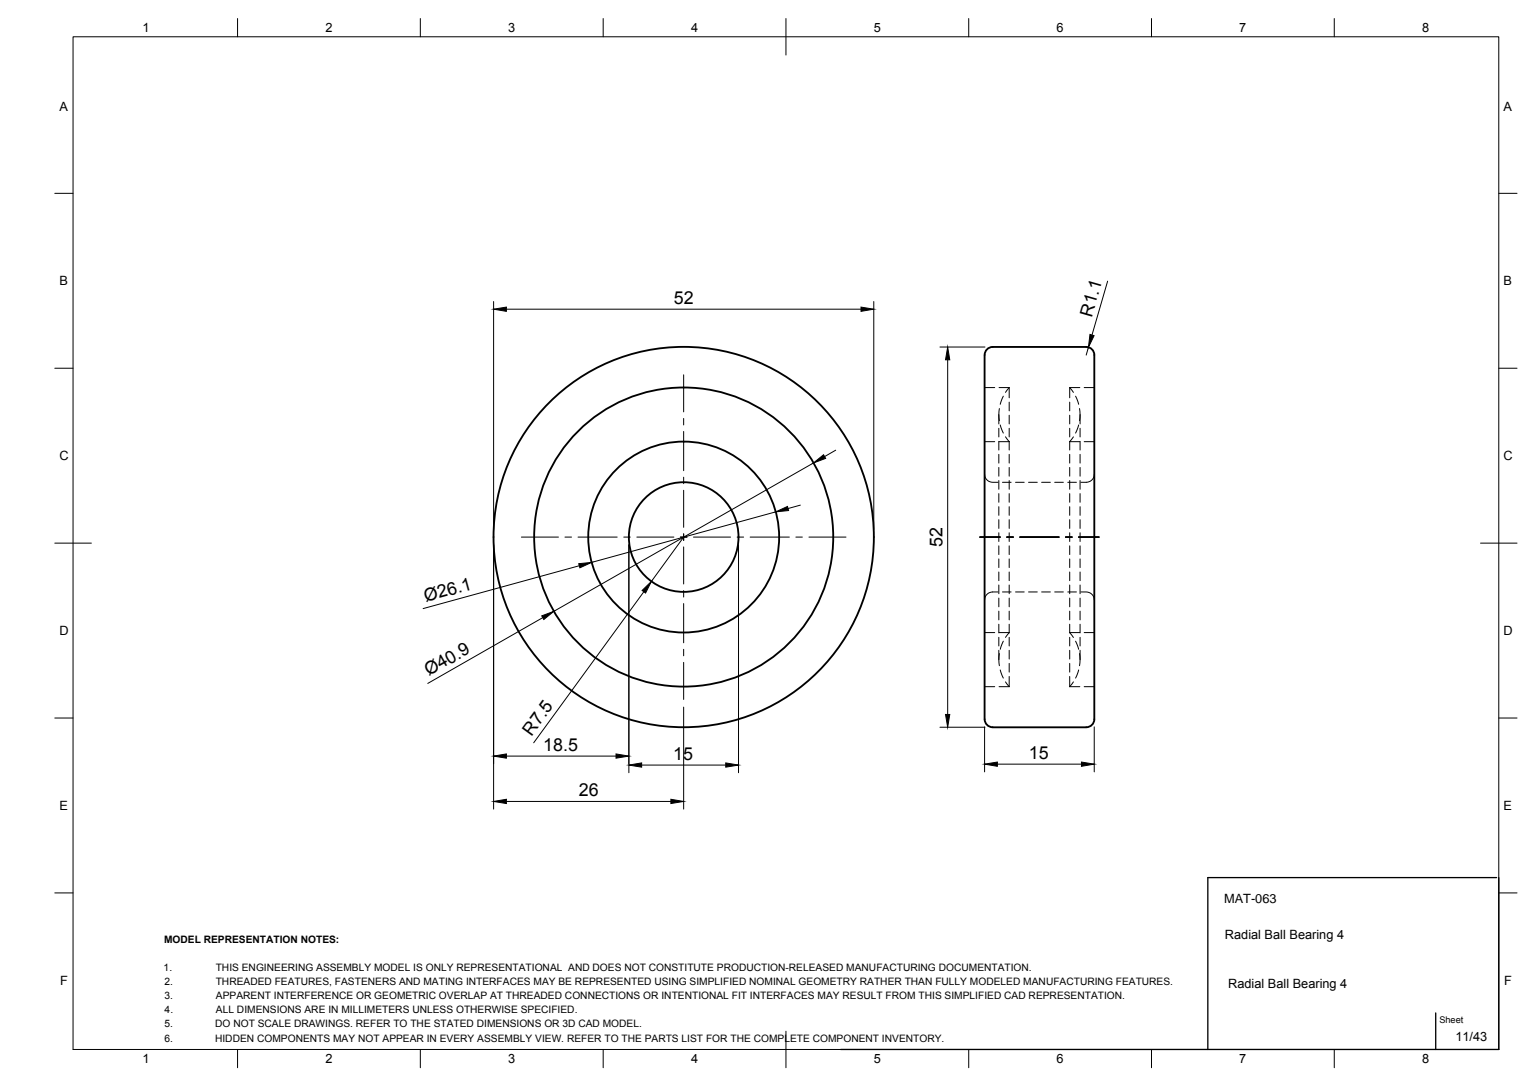
ISO-10303-21;
HEADER;
/* Generated by software containing ST-Developer
 * from STEP Tools, Inc. (www.steptools.com) 
 */

FILE_DESCRIPTION(
/* description */ (''),
/* implementation_level */ '2;1');

FILE_NAME(
/* name */ 'Radial Ball Bearing 4.step',
/* time_stamp */ '2026-10-24T09:43:01-07:00',
/* author */ (''),
/* organization */ (''),
/* preprocessor_version */ 'ST-DEVELOPER v20.2',
/* originating_system */ 'Autodesk Translation Framework v15.15.0.0',
/* authorisation */ '');

FILE_SCHEMA (('AUTOMOTIVE_DESIGN { 1 0 10303 214 3 1 1 }'));
ENDSEC;

DATA;
#10=MECHANICAL_DESIGN_GEOMETRIC_PRESENTATION_REPRESENTATION('',(#281),#11112);
#197=TOROIDAL_SURFACE('',#6769,0.0248999989285722,0.00110000131901909);
#198=TOROIDAL_SURFACE('',#6774,0.0248999989285722,0.00110000131901909);
#199=TOROIDAL_SURFACE('',#6782,0.0248999989285722,0.00110000131901911);
#200=TOROIDAL_SURFACE('',#6789,0.0248999989285722,0.00110000131901911);
#201=TOROIDAL_SURFACE('',#6793,0.01675,0.00555000054498457);
#202=TOROIDAL_SURFACE('',#6802,0.01675,0.00555000054498457);
#203=TOROIDAL_SURFACE('',#6811,0.00860000107142784,0.00110000131901912);
#204=TOROIDAL_SURFACE('',#6815,0.00860000107142784,0.00110000131901912);
#205=TOROIDAL_SURFACE('',#6823,0.00860000107142785,0.00110000131901912);
#206=TOROIDAL_SURFACE('',#6826,0.00860000107142785,0.00110000131901912);
#215=SHAPE_REPRESENTATION_RELATIONSHIP('SRR','None',#11238,#248);
#248=ADVANCED_BREP_SHAPE_REPRESENTATION('',(#314),#11083);
#281=STYLED_ITEM('',(#11425),#314);
#314=MANIFOLD_SOLID_BREP('Radial Ball Bearing 4',#6018);
#408=FACE_BOUND('',#1254,.T.);
#409=FACE_BOUND('',#1259,.T.);
#410=FACE_BOUND('',#1265,.T.);
#411=FACE_BOUND('',#1270,.T.);
#539=PLANE('',#6780);
#540=PLANE('',#6791);
#541=PLANE('',#6806);
#542=PLANE('',#6817);
#817=FACE_OUTER_BOUND('',#1250,.T.);
#818=FACE_OUTER_BOUND('',#1251,.T.);
#819=FACE_OUTER_BOUND('',#1252,.T.);
#820=FACE_OUTER_BOUND('',#1253,.T.);
#821=FACE_OUTER_BOUND('',#1255,.T.);
#822=FACE_OUTER_BOUND('',#1256,.T.);
#823=FACE_OUTER_BOUND('',#1257,.T.);
#824=FACE_OUTER_BOUND('',#1258,.T.);
#825=FACE_OUTER_BOUND('',#1260,.T.);
#826=FACE_OUTER_BOUND('',#1261,.T.);
#827=FACE_OUTER_BOUND('',#1262,.T.);
#828=FACE_OUTER_BOUND('',#1263,.T.);
#829=FACE_OUTER_BOUND('',#1264,.T.);
#830=FACE_OUTER_BOUND('',#1266,.T.);
#831=FACE_OUTER_BOUND('',#1267,.T.);
#832=FACE_OUTER_BOUND('',#1268,.T.);
#833=FACE_OUTER_BOUND('',#1269,.T.);
#834=FACE_OUTER_BOUND('',#1271,.T.);
#835=FACE_OUTER_BOUND('',#1272,.T.);
#836=FACE_OUTER_BOUND('',#1273,.T.);
#1250=EDGE_LOOP('',(#4579,#4580,#4581,#4582));
#1251=EDGE_LOOP('',(#4583,#4584,#4585,#4586));
#1252=EDGE_LOOP('',(#4587,#4588,#4589,#4590,#4591,#4592));
#1253=EDGE_LOOP('',(#4593,#4594));
#1254=EDGE_LOOP('',(#4595));
#1255=EDGE_LOOP('',(#4596,#4597,#4598,#4599));
#1256=EDGE_LOOP('',(#4600,#4601,#4602,#4603,#4604));
#1257=EDGE_LOOP('',(#4605,#4606,#4607,#4608));
#1258=EDGE_LOOP('',(#4609,#4610));
#1259=EDGE_LOOP('',(#4611));
#1260=EDGE_LOOP('',(#4612,#4613,#4614,#4615,#4616,#4617));
#1261=EDGE_LOOP('',(#4618,#4619,#4620,#4621,#4622));
#1262=EDGE_LOOP('',(#4623,#4624,#4625,#4626,#4627));
#1263=EDGE_LOOP('',(#4628,#4629,#4630,#4631,#4632,#4633));
#1264=EDGE_LOOP('',(#4634));
#1265=EDGE_LOOP('',(#4635,#4636));
#1266=EDGE_LOOP('',(#4637,#4638,#4639,#4640,#4641));
#1267=EDGE_LOOP('',(#4642,#4643,#4644,#4645));
#1268=EDGE_LOOP('',(#4646,#4647,#4648,#4649));
#1269=EDGE_LOOP('',(#4650));
#1270=EDGE_LOOP('',(#4651,#4652));
#1271=EDGE_LOOP('',(#4653,#4654,#4655,#4656,#4657,#4658));
#1272=EDGE_LOOP('',(#4659,#4660,#4661,#4662));
#1273=EDGE_LOOP('',(#4663,#4664,#4665,#4666));
#1663=LINE('',#10007,#2022);
#1664=LINE('',#10019,#2023);
#1665=LINE('',#10039,#2024);
#1666=LINE('',#10042,#2025);
#1667=LINE('',#10058,#2026);
#1668=LINE('',#10074,#2027);
#2022=VECTOR('',#8111,0.026);
#2023=VECTOR('',#8126,0.02045);
#2024=VECTOR('',#8153,0.02045);
#2025=VECTOR('',#8156,0.01305);
#2026=VECTOR('',#8177,0.01305);
#2027=VECTOR('',#8198,0.0075);
#2484=CIRCLE('',#6770,0.0248999997701383);
#2485=CIRCLE('',#6771,0.00110000131901909);
#2486=CIRCLE('',#6772,0.0260000002475909);
#2487=CIRCLE('',#6773,0.00110000131901909);
#2488=CIRCLE('',#6775,0.0248999997701383);
#2489=CIRCLE('',#6776,0.0260000002475909);
#2490=CIRCLE('',#6778,0.026);
#2491=CIRCLE('',#6779,0.026);
#2492=CIRCLE('',#6781,0.02045);
#2493=CIRCLE('',#6783,0.00110000131901911);
#2494=CIRCLE('',#6784,0.0248999997701383);
#2495=CIRCLE('',#6785,0.0011000013190191);
#2496=CIRCLE('',#6787,0.02045);
#2497=CIRCLE('',#6788,0.02045);
#2498=CIRCLE('',#6790,0.0248999997701383);
#2499=CIRCLE('',#6792,0.02045);
#2500=CIRCLE('',#6794,0.00555000054498457);
#2501=CIRCLE('',#6795,0.0130499999271107);
#2502=CIRCLE('',#6796,0.0130499999271107);
#2503=CIRCLE('',#6798,0.02045);
#2504=CIRCLE('',#6799,0.02045);
#2505=CIRCLE('',#6801,0.01305);
#2506=CIRCLE('',#6803,0.01305);
#2507=CIRCLE('',#6804,0.00555000054498457);
#2508=CIRCLE('',#6805,0.01305);
#2509=CIRCLE('',#6807,0.00860000022986177);
#2510=CIRCLE('',#6808,0.00860000022986177);
#2511=CIRCLE('',#6810,0.01305);
#2512=CIRCLE('',#6812,0.00110000131901912);
#2513=CIRCLE('',#6813,0.00749999975240907);
#2514=CIRCLE('',#6814,0.00110000131901912);
#2515=CIRCLE('',#6816,0.00749999975240873);
#2516=CIRCLE('',#6818,0.00860000022986177);
#2517=CIRCLE('',#6819,0.00860000022986177);
#2518=CIRCLE('',#6821,0.0075);
#2519=CIRCLE('',#6822,0.00749999975240873);
#2520=CIRCLE('',#6824,0.00110000131901912);
#2521=CIRCLE('',#6825,0.00110000131901912);
#2880=VERTEX_POINT('',#9991);
#2881=VERTEX_POINT('',#9992);
#2882=VERTEX_POINT('',#9994);
#2883=VERTEX_POINT('',#9996);
#2884=VERTEX_POINT('',#10003);
#2885=VERTEX_POINT('',#10004);
#2886=VERTEX_POINT('',#10009);
#2887=VERTEX_POINT('',#10012);
#2888=VERTEX_POINT('',#10014);
#2889=VERTEX_POINT('',#10018);
#2890=VERTEX_POINT('',#10020);
#2891=VERTEX_POINT('',#10026);
#2892=VERTEX_POINT('',#10029);
#2893=VERTEX_POINT('',#10031);
#2894=VERTEX_POINT('',#10035);
#2895=VERTEX_POINT('',#10036);
#2896=VERTEX_POINT('',#10041);
#2897=VERTEX_POINT('',#10045);
#2898=VERTEX_POINT('',#10046);
#2899=VERTEX_POINT('',#10051);
#2900=VERTEX_POINT('',#10052);
#2901=VERTEX_POINT('',#10056);
#2902=VERTEX_POINT('',#10060);
#2903=VERTEX_POINT('',#10062);
#2904=VERTEX_POINT('',#10068);
#2905=VERTEX_POINT('',#10069);
#2906=VERTEX_POINT('',#10073);
#2907=VERTEX_POINT('',#10075);
#3493=EDGE_CURVE('',#2880,#2881,#2484,.T.);
#3494=EDGE_CURVE('',#2881,#2882,#2485,.T.);
#3495=EDGE_CURVE('',#2882,#2883,#2486,.F.);
#3496=EDGE_CURVE('',#2883,#2880,#2487,.T.);
#3497=EDGE_CURVE('',#2881,#2880,#2488,.T.);
#3498=EDGE_CURVE('',#2883,#2882,#2489,.T.);
#3499=EDGE_CURVE('',#2884,#2885,#2490,.F.);
#3500=EDGE_CURVE('',#2885,#2884,#2491,.F.);
#3501=EDGE_CURVE('',#2884,#2882,#1663,.T.);
#3502=EDGE_CURVE('',#2886,#2886,#2492,.T.);
#3503=EDGE_CURVE('',#2884,#2887,#2493,.T.);
#3504=EDGE_CURVE('',#2887,#2888,#2494,.F.);
#3505=EDGE_CURVE('',#2888,#2885,#2495,.T.);
#3506=EDGE_CURVE('',#2886,#2889,#1664,.T.);
#3507=EDGE_CURVE('',#2890,#2889,#2496,.F.);
#3508=EDGE_CURVE('',#2889,#2890,#2497,.F.);
#3509=EDGE_CURVE('',#2888,#2887,#2498,.F.);
#3510=EDGE_CURVE('',#2891,#2891,#2499,.F.);
#3511=EDGE_CURVE('',#2890,#2892,#2500,.T.);
#3512=EDGE_CURVE('',#2892,#2893,#2501,.T.);
#3513=EDGE_CURVE('',#2893,#2892,#2502,.T.);
#3514=EDGE_CURVE('',#2894,#2895,#2503,.F.);
#3515=EDGE_CURVE('',#2895,#2894,#2504,.F.);
#3516=EDGE_CURVE('',#2895,#2891,#1665,.T.);
#3517=EDGE_CURVE('',#2893,#2896,#1666,.T.);
#3518=EDGE_CURVE('',#2896,#2896,#2505,.T.);
#3519=EDGE_CURVE('',#2897,#2898,#2506,.T.);
#3520=EDGE_CURVE('',#2898,#2894,#2507,.T.);
#3521=EDGE_CURVE('',#2898,#2897,#2508,.T.);
#3522=EDGE_CURVE('',#2899,#2900,#2509,.T.);
#3523=EDGE_CURVE('',#2900,#2899,#2510,.T.);
#3524=EDGE_CURVE('',#2901,#2901,#2511,.F.);
#3525=EDGE_CURVE('',#2901,#2897,#1667,.T.);
#3526=EDGE_CURVE('',#2900,#2902,#2512,.T.);
#3527=EDGE_CURVE('',#2902,#2903,#2513,.T.);
#3528=EDGE_CURVE('',#2903,#2899,#2514,.T.);
#3529=EDGE_CURVE('',#2903,#2902,#2515,.T.);
#3530=EDGE_CURVE('',#2904,#2905,#2516,.F.);
#3531=EDGE_CURVE('',#2905,#2904,#2517,.F.);
#3532=EDGE_CURVE('',#2902,#2906,#1668,.T.);
#3533=EDGE_CURVE('',#2907,#2906,#2518,.F.);
#3534=EDGE_CURVE('',#2906,#2907,#2519,.F.);
#3535=EDGE_CURVE('',#2906,#2904,#2520,.T.);
#3536=EDGE_CURVE('',#2905,#2907,#2521,.T.);
#4579=ORIENTED_EDGE('',*,*,#3493,.T.);
#4580=ORIENTED_EDGE('',*,*,#3494,.T.);
#4581=ORIENTED_EDGE('',*,*,#3495,.T.);
#4582=ORIENTED_EDGE('',*,*,#3496,.T.);
#4583=ORIENTED_EDGE('',*,*,#3494,.F.);
#4584=ORIENTED_EDGE('',*,*,#3497,.T.);
#4585=ORIENTED_EDGE('',*,*,#3496,.F.);
#4586=ORIENTED_EDGE('',*,*,#3498,.T.);
#4587=ORIENTED_EDGE('',*,*,#3499,.T.);
#4588=ORIENTED_EDGE('',*,*,#3500,.T.);
#4589=ORIENTED_EDGE('',*,*,#3501,.T.);
#4590=ORIENTED_EDGE('',*,*,#3498,.F.);
#4591=ORIENTED_EDGE('',*,*,#3495,.F.);
#4592=ORIENTED_EDGE('',*,*,#3501,.F.);
#4593=ORIENTED_EDGE('',*,*,#3493,.F.);
#4594=ORIENTED_EDGE('',*,*,#3497,.F.);
#4595=ORIENTED_EDGE('',*,*,#3502,.T.);
#4596=ORIENTED_EDGE('',*,*,#3499,.F.);
#4597=ORIENTED_EDGE('',*,*,#3503,.T.);
#4598=ORIENTED_EDGE('',*,*,#3504,.T.);
#4599=ORIENTED_EDGE('',*,*,#3505,.T.);
#4600=ORIENTED_EDGE('',*,*,#3502,.F.);
#4601=ORIENTED_EDGE('',*,*,#3506,.T.);
#4602=ORIENTED_EDGE('',*,*,#3507,.F.);
#4603=ORIENTED_EDGE('',*,*,#3508,.F.);
#4604=ORIENTED_EDGE('',*,*,#3506,.F.);
#4605=ORIENTED_EDGE('',*,*,#3503,.F.);
#4606=ORIENTED_EDGE('',*,*,#3500,.F.);
#4607=ORIENTED_EDGE('',*,*,#3505,.F.);
#4608=ORIENTED_EDGE('',*,*,#3509,.T.);
#4609=ORIENTED_EDGE('',*,*,#3504,.F.);
#4610=ORIENTED_EDGE('',*,*,#3509,.F.);
#4611=ORIENTED_EDGE('',*,*,#3510,.T.);
#4612=ORIENTED_EDGE('',*,*,#3508,.T.);
#4613=ORIENTED_EDGE('',*,*,#3511,.T.);
#4614=ORIENTED_EDGE('',*,*,#3512,.T.);
#4615=ORIENTED_EDGE('',*,*,#3513,.T.);
#4616=ORIENTED_EDGE('',*,*,#3511,.F.);
#4617=ORIENTED_EDGE('',*,*,#3507,.T.);
#4618=ORIENTED_EDGE('',*,*,#3514,.F.);
#4619=ORIENTED_EDGE('',*,*,#3515,.F.);
#4620=ORIENTED_EDGE('',*,*,#3516,.T.);
#4621=ORIENTED_EDGE('',*,*,#3510,.F.);
#4622=ORIENTED_EDGE('',*,*,#3516,.F.);
#4623=ORIENTED_EDGE('',*,*,#3513,.F.);
#4624=ORIENTED_EDGE('',*,*,#3517,.T.);
#4625=ORIENTED_EDGE('',*,*,#3518,.T.);
#4626=ORIENTED_EDGE('',*,*,#3517,.F.);
#4627=ORIENTED_EDGE('',*,*,#3512,.F.);
#4628=ORIENTED_EDGE('',*,*,#3519,.T.);
#4629=ORIENTED_EDGE('',*,*,#3520,.T.);
#4630=ORIENTED_EDGE('',*,*,#3514,.T.);
#4631=ORIENTED_EDGE('',*,*,#3515,.T.);
#4632=ORIENTED_EDGE('',*,*,#3520,.F.);
#4633=ORIENTED_EDGE('',*,*,#3521,.T.);
#4634=ORIENTED_EDGE('',*,*,#3518,.F.);
#4635=ORIENTED_EDGE('',*,*,#3522,.T.);
#4636=ORIENTED_EDGE('',*,*,#3523,.T.);
#4637=ORIENTED_EDGE('',*,*,#3524,.T.);
#4638=ORIENTED_EDGE('',*,*,#3525,.T.);
#4639=ORIENTED_EDGE('',*,*,#3521,.F.);
#4640=ORIENTED_EDGE('',*,*,#3519,.F.);
#4641=ORIENTED_EDGE('',*,*,#3525,.F.);
#4642=ORIENTED_EDGE('',*,*,#3526,.T.);
#4643=ORIENTED_EDGE('',*,*,#3527,.T.);
#4644=ORIENTED_EDGE('',*,*,#3528,.T.);
#4645=ORIENTED_EDGE('',*,*,#3523,.F.);
#4646=ORIENTED_EDGE('',*,*,#3529,.T.);
#4647=ORIENTED_EDGE('',*,*,#3526,.F.);
#4648=ORIENTED_EDGE('',*,*,#3522,.F.);
#4649=ORIENTED_EDGE('',*,*,#3528,.F.);
#4650=ORIENTED_EDGE('',*,*,#3524,.F.);
#4651=ORIENTED_EDGE('',*,*,#3530,.T.);
#4652=ORIENTED_EDGE('',*,*,#3531,.T.);
#4653=ORIENTED_EDGE('',*,*,#3527,.F.);
#4654=ORIENTED_EDGE('',*,*,#3532,.T.);
#4655=ORIENTED_EDGE('',*,*,#3533,.F.);
#4656=ORIENTED_EDGE('',*,*,#3534,.F.);
#4657=ORIENTED_EDGE('',*,*,#3532,.F.);
#4658=ORIENTED_EDGE('',*,*,#3529,.F.);
#4659=ORIENTED_EDGE('',*,*,#3535,.T.);
#4660=ORIENTED_EDGE('',*,*,#3531,.F.);
#4661=ORIENTED_EDGE('',*,*,#3536,.T.);
#4662=ORIENTED_EDGE('',*,*,#3533,.T.);
#4663=ORIENTED_EDGE('',*,*,#3530,.F.);
#4664=ORIENTED_EDGE('',*,*,#3535,.F.);
#4665=ORIENTED_EDGE('',*,*,#3534,.T.);
#4666=ORIENTED_EDGE('',*,*,#3536,.F.);
#5562=CYLINDRICAL_SURFACE('',#6777,0.026);
#5563=CYLINDRICAL_SURFACE('',#6786,0.02045);
#5564=CYLINDRICAL_SURFACE('',#6797,0.02045);
#5565=CYLINDRICAL_SURFACE('',#6800,0.01305);
#5566=CYLINDRICAL_SURFACE('',#6809,0.01305);
#5567=CYLINDRICAL_SURFACE('',#6820,0.0075);
#5790=ADVANCED_FACE('',(#817),#197,.T.);
#5791=ADVANCED_FACE('',(#818),#198,.T.);
#5792=ADVANCED_FACE('',(#819),#5562,.T.);
#5793=ADVANCED_FACE('',(#820,#408),#539,.T.);
#5794=ADVANCED_FACE('',(#821),#199,.T.);
#5795=ADVANCED_FACE('',(#822),#5563,.F.);
#5796=ADVANCED_FACE('',(#823),#200,.T.);
#5797=ADVANCED_FACE('',(#824,#409),#540,.T.);
#5798=ADVANCED_FACE('',(#825),#201,.T.);
#5799=ADVANCED_FACE('',(#826),#5564,.F.);
#5800=ADVANCED_FACE('',(#827),#5565,.T.);
#5801=ADVANCED_FACE('',(#828),#202,.T.);
#5802=ADVANCED_FACE('',(#829,#410),#541,.T.);
#5803=ADVANCED_FACE('',(#830),#5566,.T.);
#5804=ADVANCED_FACE('',(#831),#203,.T.);
#5805=ADVANCED_FACE('',(#832),#204,.T.);
#5806=ADVANCED_FACE('',(#833,#411),#542,.T.);
#5807=ADVANCED_FACE('',(#834),#5567,.F.);
#5808=ADVANCED_FACE('',(#835),#205,.T.);
#5809=ADVANCED_FACE('',(#836),#206,.T.);
#6018=CLOSED_SHELL('',(#5790,#5791,#5792,#5793,#5794,#5795,#5796,#5797,
#5798,#5799,#5800,#5801,#5802,#5803,#5804,#5805,#5806,#5807,#5808,#5809));
#6768=AXIS2_PLACEMENT_3D('',#9989,#8087,#8088);
#6769=AXIS2_PLACEMENT_3D('',#9990,#8089,#8090);
#6770=AXIS2_PLACEMENT_3D('',#9993,#8091,#8092);
#6771=AXIS2_PLACEMENT_3D('',#9995,#8093,#8094);
#6772=AXIS2_PLACEMENT_3D('',#9997,#8095,#8096);
#6773=AXIS2_PLACEMENT_3D('',#9998,#8097,#8098);
#6774=AXIS2_PLACEMENT_3D('',#9999,#8099,#8100);
#6775=AXIS2_PLACEMENT_3D('',#10000,#8101,#8102);
#6776=AXIS2_PLACEMENT_3D('',#10001,#8103,#8104);
#6777=AXIS2_PLACEMENT_3D('',#10002,#8105,#8106);
#6778=AXIS2_PLACEMENT_3D('',#10005,#8107,#8108);
#6779=AXIS2_PLACEMENT_3D('',#10006,#8109,#8110);
#6780=AXIS2_PLACEMENT_3D('',#10008,#8112,#8113);
#6781=AXIS2_PLACEMENT_3D('',#10010,#8114,#8115);
#6782=AXIS2_PLACEMENT_3D('',#10011,#8116,#8117);
#6783=AXIS2_PLACEMENT_3D('',#10013,#8118,#8119);
#6784=AXIS2_PLACEMENT_3D('',#10015,#8120,#8121);
#6785=AXIS2_PLACEMENT_3D('',#10016,#8122,#8123);
#6786=AXIS2_PLACEMENT_3D('',#10017,#8124,#8125);
#6787=AXIS2_PLACEMENT_3D('',#10021,#8127,#8128);
#6788=AXIS2_PLACEMENT_3D('',#10022,#8129,#8130);
#6789=AXIS2_PLACEMENT_3D('',#10023,#8131,#8132);
#6790=AXIS2_PLACEMENT_3D('',#10024,#8133,#8134);
#6791=AXIS2_PLACEMENT_3D('',#10025,#8135,#8136);
#6792=AXIS2_PLACEMENT_3D('',#10027,#8137,#8138);
#6793=AXIS2_PLACEMENT_3D('',#10028,#8139,#8140);
#6794=AXIS2_PLACEMENT_3D('',#10030,#8141,#8142);
#6795=AXIS2_PLACEMENT_3D('',#10032,#8143,#8144);
#6796=AXIS2_PLACEMENT_3D('',#10033,#8145,#8146);
#6797=AXIS2_PLACEMENT_3D('',#10034,#8147,#8148);
#6798=AXIS2_PLACEMENT_3D('',#10037,#8149,#8150);
#6799=AXIS2_PLACEMENT_3D('',#10038,#8151,#8152);
#6800=AXIS2_PLACEMENT_3D('',#10040,#8154,#8155);
#6801=AXIS2_PLACEMENT_3D('',#10043,#8157,#8158);
#6802=AXIS2_PLACEMENT_3D('',#10044,#8159,#8160);
#6803=AXIS2_PLACEMENT_3D('',#10047,#8161,#8162);
#6804=AXIS2_PLACEMENT_3D('',#10048,#8163,#8164);
#6805=AXIS2_PLACEMENT_3D('',#10049,#8165,#8166);
#6806=AXIS2_PLACEMENT_3D('',#10050,#8167,#8168);
#6807=AXIS2_PLACEMENT_3D('',#10053,#8169,#8170);
#6808=AXIS2_PLACEMENT_3D('',#10054,#8171,#8172);
#6809=AXIS2_PLACEMENT_3D('',#10055,#8173,#8174);
#6810=AXIS2_PLACEMENT_3D('',#10057,#8175,#8176);
#6811=AXIS2_PLACEMENT_3D('',#10059,#8178,#8179);
#6812=AXIS2_PLACEMENT_3D('',#10061,#8180,#8181);
#6813=AXIS2_PLACEMENT_3D('',#10063,#8182,#8183);
#6814=AXIS2_PLACEMENT_3D('',#10064,#8184,#8185);
#6815=AXIS2_PLACEMENT_3D('',#10065,#8186,#8187);
#6816=AXIS2_PLACEMENT_3D('',#10066,#8188,#8189);
#6817=AXIS2_PLACEMENT_3D('',#10067,#8190,#8191);
#6818=AXIS2_PLACEMENT_3D('',#10070,#8192,#8193);
#6819=AXIS2_PLACEMENT_3D('',#10071,#8194,#8195);
#6820=AXIS2_PLACEMENT_3D('',#10072,#8196,#8197);
#6821=AXIS2_PLACEMENT_3D('',#10076,#8199,#8200);
#6822=AXIS2_PLACEMENT_3D('',#10077,#8201,#8202);
#6823=AXIS2_PLACEMENT_3D('',#10078,#8203,#8204);
#6824=AXIS2_PLACEMENT_3D('',#10079,#8205,#8206);
#6825=AXIS2_PLACEMENT_3D('',#10080,#8207,#8208);
#6826=AXIS2_PLACEMENT_3D('',#10081,#8209,#8210);
#8087=DIRECTION('axis',(0.,0.,1.));
#8088=DIRECTION('refdir',(1.,0.,0.));
#8089=DIRECTION('center_axis',(1.,4.17203717831812E-9,1.01277540341552E-17));
#8090=DIRECTION('ref_axis',(-4.1720371751696E-9,1.,0.));
#8091=DIRECTION('center_axis',(1.,4.17203717831812E-9,1.01277540341552E-17));
#8092=DIRECTION('ref_axis',(-4.17203717831812E-9,1.,-1.69634196247466E-42));
#8093=DIRECTION('center_axis',(8.36866394062756E-10,1.,-8.36884415538179E-10));
#8094=DIRECTION('ref_axis',(-7.96162761077703E-7,8.36885081819775E-10,0.999999999999683));
#8095=DIRECTION('center_axis',(1.,4.17203717831812E-9,1.01277540341552E-17));
#8096=DIRECTION('ref_axis',(-4.17203717831812E-9,1.,-1.69634196247466E-42));
#8097=DIRECTION('center_axis',(8.36869948186391E-10,1.,8.36891441629708E-10));
#8098=DIRECTION('ref_axis',(-0.999999999999707,8.36870588457614E-10,-7.65059166582913E-7));
#8099=DIRECTION('center_axis',(1.,-4.17203708245403E-9,6.73890284431642E-18));
#8100=DIRECTION('ref_axis',(-4.1720370750894E-9,-1.,5.66553889764798E-16));
#8101=DIRECTION('center_axis',(1.,-4.17203708245403E-9,6.73890284431642E-18));
#8102=DIRECTION('ref_axis',(4.17203708245403E-9,1.,-1.23465054354127E-43));
#8103=DIRECTION('center_axis',(-1.,4.17203697154146E-9,4.27849718847752E-19));
#8104=DIRECTION('ref_axis',(-4.27008851558771E-17,-5.34839554841822E-9,
1.));
#8105=DIRECTION('center_axis',(1.,0.,-3.33600668457079E-17));
#8106=DIRECTION('ref_axis',(-3.33600668457079E-17,0.,-1.));
#8107=DIRECTION('center_axis',(1.,0.,-3.33600668457079E-17));
#8108=DIRECTION('ref_axis',(-3.33600668457079E-17,0.,-1.));
#8109=DIRECTION('center_axis',(1.,0.,0.));
#8110=DIRECTION('ref_axis',(0.,-4.64793894161955E-10,-1.));
#8111=DIRECTION('',(-1.,0.,3.33600668457079E-17));
#8112=DIRECTION('center_axis',(-1.,1.53144334479515E-17,1.9842828066192E-17));
#8113=DIRECTION('ref_axis',(1.9842828066192E-17,0.,1.));
#8114=DIRECTION('center_axis',(1.,0.,0.));
#8115=DIRECTION('ref_axis',(0.,0.,-1.));
#8116=DIRECTION('center_axis',(1.,-4.17203727418451E-9,-1.07069540457721E-17));
#8117=DIRECTION('ref_axis',(4.1720372752498E-9,1.,0.));
#8118=DIRECTION('center_axis',(-8.36866342496331E-10,1.,-8.36883936494317E-10));
#8119=DIRECTION('ref_axis',(0.999999999999707,8.36866982761818E-10,7.65059174657239E-7));
#8120=DIRECTION('center_axis',(1.,-4.17203727418451E-9,-1.07069540457721E-17));
#8121=DIRECTION('ref_axis',(4.17203727418451E-9,1.,1.45967462857766E-42));
#8122=DIRECTION('center_axis',(-8.36844869453255E-10,1.,8.36865935422119E-10));
#8123=DIRECTION('ref_axis',(9.00645352209864E-7,8.36866689122222E-10,-0.999999999999595));
#8124=DIRECTION('center_axis',(1.,0.,0.));
#8125=DIRECTION('ref_axis',(0.,0.,-1.));
#8126=DIRECTION('',(1.,0.,0.));
#8127=DIRECTION('center_axis',(1.,0.,0.));
#8128=DIRECTION('ref_axis',(0.,-4.29586394988857E-10,-1.));
#8129=DIRECTION('center_axis',(1.,0.,0.));
#8130=DIRECTION('ref_axis',(0.,-4.29586394988857E-10,-1.));
#8131=DIRECTION('center_axis',(1.,4.17203725971588E-9,2.0031116033889E-18));
#8132=DIRECTION('ref_axis',(4.1720372752498E-9,-1.,5.66553889764798E-16));
#8133=DIRECTION('center_axis',(1.,4.17203725971588E-9,2.0031116033889E-18));
#8134=DIRECTION('ref_axis',(-4.17203725971588E-9,1.,5.39459847610519E-43));
#8135=DIRECTION('center_axis',(1.,1.53144334479515E-17,-1.9842828066192E-17));
#8136=DIRECTION('ref_axis',(-1.9842828066192E-17,0.,-1.));
#8137=DIRECTION('center_axis',(1.,0.,0.));
#8138=DIRECTION('ref_axis',(0.,0.,-1.));
#8139=DIRECTION('center_axis',(1.,6.36556116938371E-17,1.00386354793954E-17));
#8140=DIRECTION('ref_axis',(-6.3655612933414E-17,1.,0.));
#8141=DIRECTION('center_axis',(1.00386354793954E-17,1.22464679914735E-16,
-1.));
#8142=DIRECTION('ref_axis',(6.36556105223495E-17,-1.,-1.22464679914735E-16));
#8143=DIRECTION('center_axis',(1.,1.35504238326755E-16,2.34999225611352E-17));
#8144=DIRECTION('ref_axis',(-1.35504238326755E-16,1.,1.40763492406121E-49));
#8145=DIRECTION('center_axis',(1.,1.35504238326755E-16,2.34999225611352E-17));
#8146=DIRECTION('ref_axis',(-1.35504238326755E-16,1.,1.40763492406121E-49));
#8147=DIRECTION('center_axis',(1.,0.,0.));
#8148=DIRECTION('ref_axis',(0.,0.,-1.));
#8149=DIRECTION('center_axis',(-1.,0.,0.));
#8150=DIRECTION('ref_axis',(0.,-6.60206605267583E-10,1.));
#8151=DIRECTION('center_axis',(-1.,0.,0.));
#8152=DIRECTION('ref_axis',(0.,-6.60206605267583E-10,1.));
#8153=DIRECTION('',(1.,0.,0.));
#8154=DIRECTION('center_axis',(1.,0.,0.));
#8155=DIRECTION('ref_axis',(0.,0.,-1.));
#8156=DIRECTION('',(-1.,0.,0.));
#8157=DIRECTION('center_axis',(1.,0.,0.));
#8158=DIRECTION('ref_axis',(0.,0.,-1.));
#8159=DIRECTION('center_axis',(1.,1.18552772674719E-16,-1.97711088800387E-17));
#8160=DIRECTION('ref_axis',(-1.18552772074394E-16,1.,0.));
#8161=DIRECTION('center_axis',(-1.,0.,0.));
#8162=DIRECTION('ref_axis',(0.,-2.05103586755523E-10,1.));
#8163=DIRECTION('center_axis',(-1.97711088800387E-17,1.22464679914735E-16,
-1.));
#8164=DIRECTION('ref_axis',(1.18552771796194E-16,-1.,-1.22464679914735E-16));
#8165=DIRECTION('center_axis',(-1.,0.,0.));
#8166=DIRECTION('ref_axis',(0.,-2.05103586755523E-10,1.));
#8167=DIRECTION('center_axis',(-1.,2.92206431305708E-17,3.78610282642285E-17));
#8168=DIRECTION('ref_axis',(3.78610282642285E-17,0.,1.));
#8169=DIRECTION('center_axis',(1.,1.20795004338275E-8,6.525328094131E-17));
#8170=DIRECTION('ref_axis',(-1.20795004338275E-8,1.,4.44135209129409E-41));
#8171=DIRECTION('center_axis',(1.,-1.20794999078492E-8,-6.65136044666218E-17));
#8172=DIRECTION('ref_axis',(1.20794999078492E-8,1.,-3.20659696454606E-41));
#8173=DIRECTION('center_axis',(1.,0.,0.));
#8174=DIRECTION('ref_axis',(0.,0.,-1.));
#8175=DIRECTION('center_axis',(1.,0.,0.));
#8176=DIRECTION('ref_axis',(0.,0.,-1.));
#8177=DIRECTION('',(-1.,0.,0.));
#8178=DIRECTION('center_axis',(1.,-1.20794999078492E-8,-6.65136044666218E-17));
#8179=DIRECTION('ref_axis',(-1.20794999243885E-8,-1.,-5.21792575105832E-12));
#8180=DIRECTION('center_axis',(-3.90112644891662E-10,-1.,-3.90117034748036E-10));
#8181=DIRECTION('ref_axis',(-7.96162782272821E-7,3.90117345341081E-10,-0.999999999999683));
#8182=DIRECTION('center_axis',(1.,-1.20794992145421E-8,-4.8381018443521E-19));
#8183=DIRECTION('ref_axis',(1.48029741503464E-16,1.78300800621899E-8,-1.));
#8184=DIRECTION('center_axis',(-3.90083830404282E-10,-1.,3.90119162273478E-10));
#8185=DIRECTION('ref_axis',(-0.999999999999707,3.90084128868405E-10,7.65059156489968E-7));
#8186=DIRECTION('center_axis',(1.,1.20795004338275E-8,6.525328094131E-17));
#8187=DIRECTION('ref_axis',(-1.20795004609008E-8,1.,0.));
#8188=DIRECTION('center_axis',(1.,1.20795004338275E-8,6.525328094131E-17));
#8189=DIRECTION('ref_axis',(-1.20795004338275E-8,1.,4.44135209129409E-41));
#8190=DIRECTION('center_axis',(1.,2.92206431305708E-17,-3.78610282642285E-17));
#8191=DIRECTION('ref_axis',(-3.78610282642285E-17,0.,-1.));
#8192=DIRECTION('center_axis',(1.,-1.20794999071527E-8,2.28224857621035E-17));
#8193=DIRECTION('ref_axis',(1.20794999071527E-8,1.,-1.89856639006012E-41));
#8194=DIRECTION('center_axis',(1.,1.20794999172425E-8,-1.59545740616835E-17));
#8195=DIRECTION('ref_axis',(-1.20794999172425E-8,1.,2.99570552288603E-42));
#8196=DIRECTION('center_axis',(1.,0.,-1.15648231731787E-16));
#8197=DIRECTION('ref_axis',(-1.15648231731787E-16,0.,-1.));
#8198=DIRECTION('',(1.,0.,-1.15648231731787E-16));
#8199=DIRECTION('center_axis',(1.,0.,0.));
#8200=DIRECTION('ref_axis',(0.,-4.29586131949163E-10,-1.));
#8201=DIRECTION('center_axis',(1.,-1.20794999071527E-8,2.28224857621035E-17));
#8202=DIRECTION('ref_axis',(1.20794999071527E-8,1.,-1.89856639006012E-41));
#8203=DIRECTION('center_axis',(1.,1.20794999172425E-8,-1.59545740616835E-17));
#8204=DIRECTION('ref_axis',(1.20794999243885E-8,-1.,-8.2319592183107E-12));
#8205=DIRECTION('center_axis',(3.9010897446429E-10,-1.,-3.90108144056802E-10));
#8206=DIRECTION('ref_axis',(0.999999999999707,3.90109272919983E-10,-7.65059154471383E-7));
#8207=DIRECTION('center_axis',(3.90083837031876E-10,-1.,3.90119162425402E-10));
#8208=DIRECTION('ref_axis',(7.96162783282112E-7,3.90119472995512E-10,0.999999999999683));
#8209=DIRECTION('center_axis',(1.,-1.20794999071527E-8,2.28224857621035E-17));
#8210=DIRECTION('ref_axis',(1.20794999243885E-8,1.,0.));
#9989=CARTESIAN_POINT('',(0.,0.,0.));
#9990=CARTESIAN_POINT('Origin',(-0.00639999889435817,-1.33725586897056E-10,
-2.60202312123977E-18));
#9991=CARTESIAN_POINT('',(-0.00750000021337694,-2.62982038223811E-17,-0.0248999997701383));
#9992=CARTESIAN_POINT('',(-0.00750000021337694,-9.33158505355009E-18,0.0248999997701383));
#9993=CARTESIAN_POINT('Origin',(-0.00750000021337694,-1.38314833296201E-10,
-2.61316366403604E-18));
#9994=CARTESIAN_POINT('',(-0.00639999976976533,-1.58005919577827E-12,0.0260000002475909));
#9995=CARTESIAN_POINT('Origin',(-0.00639999889435817,-9.20581548326642E-13,
0.0248999989285722));
#9996=CARTESIAN_POINT('',(-0.00639999976976533,-3.35121902792442E-17,-0.0260000002475909));
#9997=CARTESIAN_POINT('Origin',(-0.00639999977013826,-1.33725590550843E-10,
-2.60202313010945E-18));
#9998=CARTESIAN_POINT('Origin',(-0.00639999889435817,-9.20629689158185E-13,
-0.0248999989285722));
#9999=CARTESIAN_POINT('Origin',(-0.00639999889435817,1.33725588194013E-10,
-2.25687613815873E-19));
#10000=CARTESIAN_POINT('Origin',(-0.00750000021337694,1.38314834487708E-10,
-2.3310041583336E-19));
#10001=CARTESIAN_POINT('Origin',(-0.00639999977013826,1.3372558821988E-10,
4.44089209850063E-18));
#10002=CARTESIAN_POINT('Origin',(-0.0206375,0.,-4.33144407778805E-52));
#10003=CARTESIAN_POINT('',(0.00639999998722997,-6.70342338705283E-12,0.0260000000825303));
#10004=CARTESIAN_POINT('',(0.00639999998722997,-5.37097589710219E-12,-0.0260000000825303));
#10005=CARTESIAN_POINT('Origin',(0.0064,0.,-9.01972807340825E-19));
#10006=CARTESIAN_POINT('Origin',(0.0064,2.91826343292479E-18,0.));
#10007=CARTESIAN_POINT('',(-0.0206375,-3.18408167778312E-18,0.026));
#10008=CARTESIAN_POINT('Origin',(-0.0075,-1.31838984174237E-18,-1.2490009027033E-18));
#10009=CARTESIAN_POINT('',(-0.0075,-2.50440270425634E-18,0.02045));
#10010=CARTESIAN_POINT('Origin',(-0.0075,0.,0.));
#10011=CARTESIAN_POINT('Origin',(0.00639999889435816,-1.33725593635445E-10,
-3.59711256079879E-19));
#10012=CARTESIAN_POINT('',(0.00750000021337694,-1.05191955076574E-17,0.0248999997701383));
#10013=CARTESIAN_POINT('Origin',(0.00639999889435816,-9.20588335445364E-13,
0.0248999989285722));
#10014=CARTESIAN_POINT('',(0.00750000021337694,-2.93287844693988E-17,-0.0248999997701383));
#10015=CARTESIAN_POINT('Origin',(0.00750000021337694,-1.38314840140043E-10,
-3.71488919652902E-19));
#10016=CARTESIAN_POINT('Origin',(0.00639999889435816,-9.20608946339399E-13,
-0.0248999989285722));
#10017=CARTESIAN_POINT('Origin',(-0.0206375,0.,0.));
#10018=CARTESIAN_POINT('',(-0.00413672599961696,1.0458235455062E-18,0.0204500000364447));
#10019=CARTESIAN_POINT('',(-0.0206375,-2.50440270425634E-18,0.02045));
#10020=CARTESIAN_POINT('',(-0.004136726,-0.02045,-2.79956704802153E-18));
#10021=CARTESIAN_POINT('Origin',(-0.004136726,1.15025496390116E-19,8.88178419700125E-18));
#10022=CARTESIAN_POINT('Origin',(-0.004136726,1.15025496390116E-19,8.88178419700125E-18));
#10023=CARTESIAN_POINT('Origin',(0.00639999889435816,1.33725592594967E-10,
2.43522299685913E-19));
#10024=CARTESIAN_POINT('Origin',(0.00750000021337694,1.3831483908365E-10,
2.45725725091783E-19));
#10025=CARTESIAN_POINT('Origin',(0.0075,-1.31838984174237E-18,1.2490009027033E-18));
#10026=CARTESIAN_POINT('',(0.0075,-2.50440270425634E-18,0.02045));
#10027=CARTESIAN_POINT('Origin',(0.0075,0.,0.));
#10028=CARTESIAN_POINT('Origin',(4.25120033285821E-10,2.32696931299848E-18,
-2.53637255105429E-19));
#10029=CARTESIAN_POINT('',(-0.00413672599923392,-0.0130499999271107,-1.89332840771843E-18));
#10030=CARTESIAN_POINT('Origin',(4.25120034352053E-10,-0.01675,-2.30492064367725E-18));
#10031=CARTESIAN_POINT('',(-0.00413672599923392,-9.72427111671565E-12,0.0130499999635554));
#10032=CARTESIAN_POINT('Origin',(-0.00413672599923392,-2.48296911984889E-18,
-8.56610574398074E-20));
#10033=CARTESIAN_POINT('Origin',(-0.00413672599923392,-2.48296911984889E-18,
-8.56610574398074E-20));
#10034=CARTESIAN_POINT('Origin',(-0.0206375,0.,0.));
#10035=CARTESIAN_POINT('',(0.004136726,-0.02045,-1.97855791081413E-18));
#10036=CARTESIAN_POINT('',(0.004136726,-2.50440270425634E-18,0.02045));
#10037=CARTESIAN_POINT('Origin',(0.004136726,-1.49874617044541E-18,-8.88178419700125E-18));
#10038=CARTESIAN_POINT('Origin',(0.004136726,-1.49874617044541E-18,-8.88178419700125E-18));
#10039=CARTESIAN_POINT('',(-0.0206375,-2.50440270425634E-18,0.02045));
#10040=CARTESIAN_POINT('Origin',(-0.0206375,0.,0.));
#10041=CARTESIAN_POINT('',(-0.0075,-1.5981640728873E-18,0.01305));
#10042=CARTESIAN_POINT('',(-0.0206375,-1.5981640728873E-18,0.01305));
#10043=CARTESIAN_POINT('Origin',(-0.0075,0.,0.));
#10044=CARTESIAN_POINT('Origin',(-4.25120036303284E-10,3.75386134271222E-18,
6.07632462000188E-19));
#10045=CARTESIAN_POINT('',(0.00413672599923392,-2.67659699192252E-12,0.0130499999635553));
#10046=CARTESIAN_POINT('',(0.00413672599923392,-0.01305,-1.07231927942994E-18));
#10047=CARTESIAN_POINT('Origin',(0.00413672599923392,-3.3221160294436E-19,
2.22044604925031E-18));
#10048=CARTESIAN_POINT('Origin',(-4.25120034317525E-10,-0.01675,-1.44365092657163E-18));
#10049=CARTESIAN_POINT('Origin',(0.00413672599923392,-3.3221160294436E-19,
2.22044604925031E-18));
#10050=CARTESIAN_POINT('Origin',(-0.0075,-1.3010426069826E-19,-1.1666015375944E-18));
#10051=CARTESIAN_POINT('',(-0.00750000021337695,-7.32444758467801E-18,-0.00860000022986174));
#10052=CARTESIAN_POINT('',(-0.00750000021337695,-9.55563692214474E-13,0.00860000022983698));
#10053=CARTESIAN_POINT('Origin',(-0.00750000021337695,1.20438122996688E-10,
1.91155415755433E-19));
#10054=CARTESIAN_POINT('Origin',(-0.00750000021337695,-1.20438124044286E-10,
-1.263242268E-19));
#10055=CARTESIAN_POINT('Origin',(-0.0206375,0.,0.));
#10056=CARTESIAN_POINT('',(0.0075,-1.5981640728873E-18,0.01305));
#10057=CARTESIAN_POINT('Origin',(0.0075,0.,0.));
#10058=CARTESIAN_POINT('',(-0.0206375,-1.5981640728873E-18,0.01305));
#10059=CARTESIAN_POINT('Origin',(-0.00639999889435815,-1.33725589876008E-10,
-1.99489279445979E-19));
#10060=CARTESIAN_POINT('',(-0.00639999933187528,-1.78004529143068E-13,0.00749999975240887));
#10061=CARTESIAN_POINT('Origin',(-0.00639999889435815,-4.29138899262724E-13,
0.00860000107142784));
#10062=CARTESIAN_POINT('',(-0.00639999933187528,7.82593383085413E-14,-0.00749999975240887));
#10063=CARTESIAN_POINT('Origin',(-0.00639999977013826,-1.33725577217623E-10,
-2.22044604925031E-18));
#10064=CARTESIAN_POINT('Origin',(-0.00639999889435815,-4.29112928832131E-13,
-0.00860000107142784));
#10065=CARTESIAN_POINT('Origin',(-0.00639999889435816,1.33725589406987E-10,
2.62934110861178E-19));
#10066=CARTESIAN_POINT('Origin',(-0.00639999889435816,1.33725589406987E-10,
2.62934110861178E-19));
#10067=CARTESIAN_POINT('Origin',(0.0075,-1.3010426069826E-19,1.1666015375944E-18));
#10068=CARTESIAN_POINT('',(0.00750000021337695,-1.12844211802569E-18,0.00860000022986174));
#10069=CARTESIAN_POINT('',(0.00750000021337695,-9.55567354576375E-13,-0.00860000022983698));
#10070=CARTESIAN_POINT('Origin',(0.00750000021337695,1.20438122943562E-10,
-1.36910420000699E-19));
#10071=CARTESIAN_POINT('Origin',(0.00750000021337695,-1.20438123513651E-10,
2.9038238015475E-19));
#10072=CARTESIAN_POINT('Origin',(-0.0206375,0.,-2.49552314011156E-51));
#10073=CARTESIAN_POINT('',(0.00639999944717908,-3.41326938021997E-12,0.00749999987620436));
#10074=CARTESIAN_POINT('',(-0.0206375,-9.18485099360515E-19,0.0075));
#10075=CARTESIAN_POINT('',(0.00639999944670613,1.23481356905966E-13,-0.0074999998349392));
#10076=CARTESIAN_POINT('Origin',(0.0064,-1.93061231994698E-18,-5.55111512312578E-18));
#10077=CARTESIAN_POINT('Origin',(0.00639999889435815,1.33725588774518E-10,
-1.62015184442301E-19));
#10078=CARTESIAN_POINT('Origin',(0.00639999889435815,-1.33725589355705E-10,
3.07932432666985E-19));
#10079=CARTESIAN_POINT('Origin',(0.00639999889435815,-4.29128599184298E-13,
0.00860000107142785));
#10080=CARTESIAN_POINT('Origin',(0.00639999889435815,-4.2911240869608E-13,
-0.00860000107142785));
#10081=CARTESIAN_POINT('Origin',(0.00639999889435815,1.33725588774518E-10,
-1.62015184442301E-19));
#11044=UNCERTAINTY_MEASURE_WITH_UNIT(LENGTH_MEASURE(1.E-5),#11113,
'DISTANCE_ACCURACY_VALUE',
'Maximum model space distance between geometric entities at asserted c
onnectivities');
#11073=UNCERTAINTY_MEASURE_WITH_UNIT(LENGTH_MEASURE(1.E-5),#11113,
'DISTANCE_ACCURACY_VALUE',
'Maximum model space distance between geometric entities at asserted c
onnectivities');
#11083=(
GEOMETRIC_REPRESENTATION_CONTEXT(3)
GLOBAL_UNCERTAINTY_ASSIGNED_CONTEXT((#11044))
GLOBAL_UNIT_ASSIGNED_CONTEXT((#11113,#11114,#11115))
REPRESENTATION_CONTEXT('','3D')
);
#11112=(
GEOMETRIC_REPRESENTATION_CONTEXT(3)
GLOBAL_UNCERTAINTY_ASSIGNED_CONTEXT((#11073))
GLOBAL_UNIT_ASSIGNED_CONTEXT((#11113,#11114,#11115))
REPRESENTATION_CONTEXT('','3D')
);
#11113=(
LENGTH_UNIT()
NAMED_UNIT(*)
SI_UNIT($,.METRE.)
);
#11114=(
NAMED_UNIT(*)
PLANE_ANGLE_UNIT()
SI_UNIT($,.RADIAN.)
);
#11115=(
NAMED_UNIT(*)
SI_UNIT($,.STERADIAN.)
SOLID_ANGLE_UNIT()
);
#11125=SHAPE_DEFINITION_REPRESENTATION(#11163,#11238);
#11163=PRODUCT_DEFINITION_SHAPE('',$,#11277);
#11238=SHAPE_REPRESENTATION('',(#6768),#11083);
#11267=PRODUCT_DEFINITION_CONTEXT('part definition',#11383,'design');
#11277=PRODUCT_DEFINITION('Radial Ball Bearing 4',
'Radial Ball Bearing 4',#11315,#11267);
#11315=PRODUCT_DEFINITION_FORMATION('',$,#11394);
#11383=APPLICATION_CONTEXT(
'Core Data for Automotive Mechanical Design Process');
#11384=PRODUCT_CONTEXT('part definition',#11383,'mechanical');
#11394=PRODUCT('Radial Ball Bearing 4','Radial Ball Bearing 4',
'radial ball bearing_68_as_AS_ISO 15 RBB - 415 - 6,SI,NC,6_68__ DE    
10847',(#11384));
#11425=PRESENTATION_STYLE_ASSIGNMENT((#11429));
#11429=SURFACE_STYLE_USAGE(.BOTH.,#11433);
#11433=SURFACE_SIDE_STYLE('',(#11437));
#11437=SURFACE_STYLE_FILL_AREA(#11441);
#11441=FILL_AREA_STYLE('Opaque(255,242,232)',(#11445));
#11445=FILL_AREA_STYLE_COLOUR('Opaque(255,242,232)',#11449);
#11449=COLOUR_RGB('Opaque(255,242,232)',1.,0.949019607843137,0.909803921568627);
ENDSEC;
END-ISO-10303-21;
